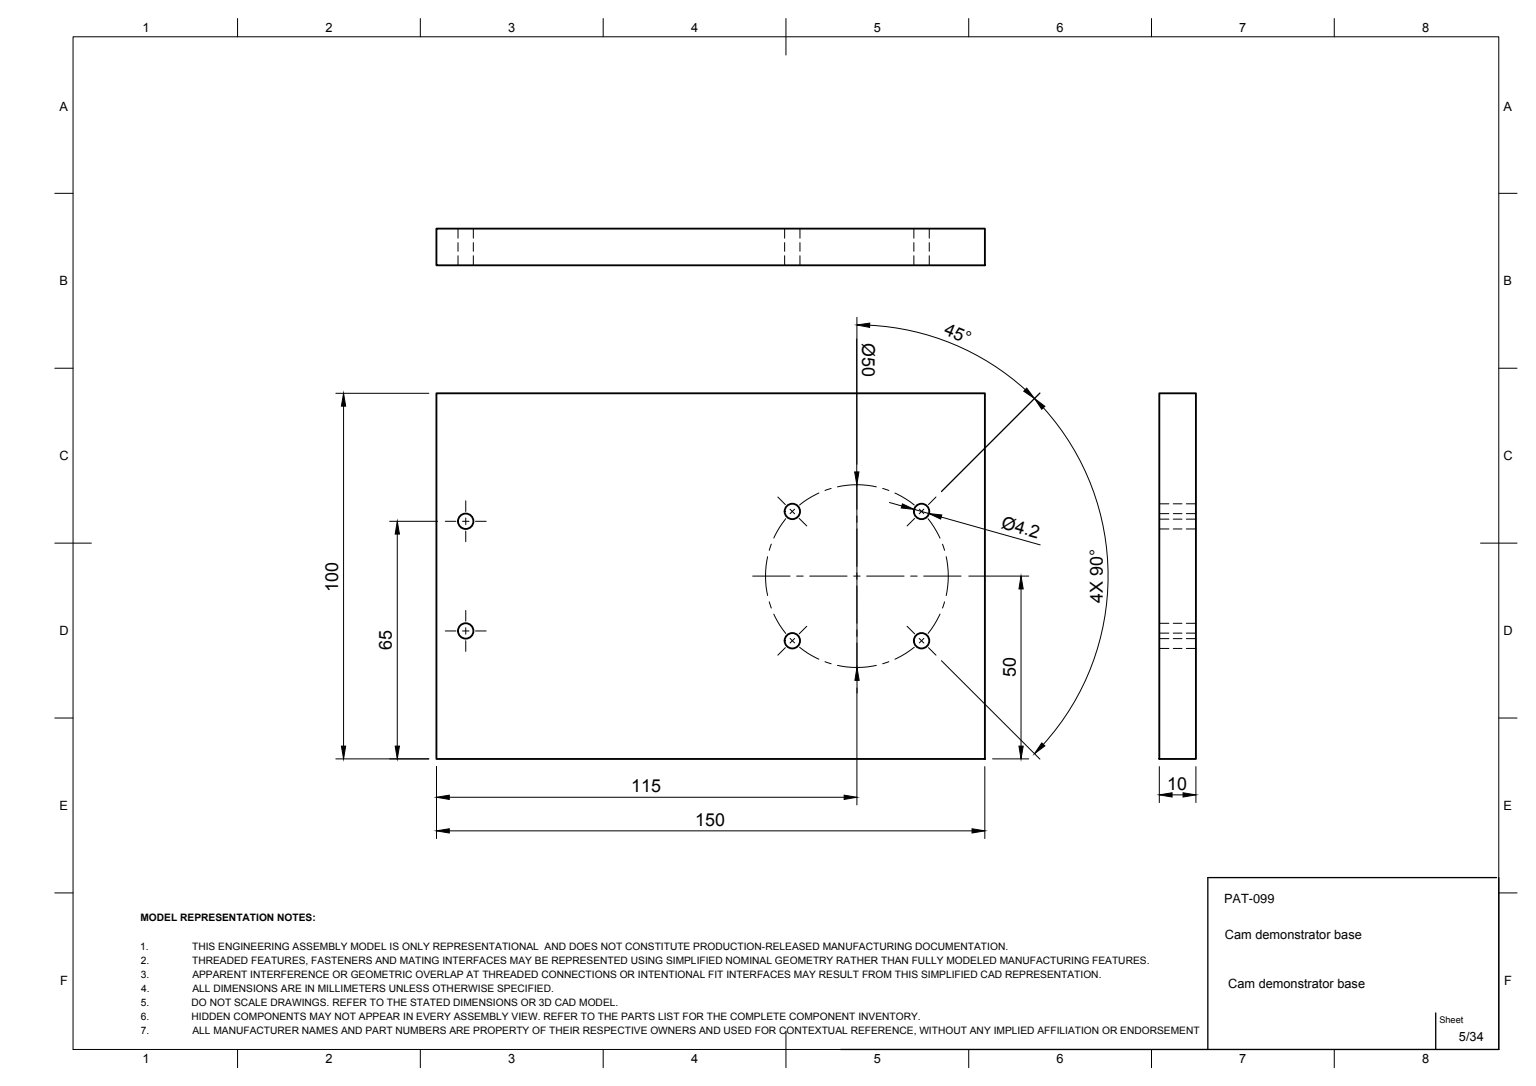
ISO-10303-21;
HEADER;
/* Generated by software containing ST-Developer
 * from STEP Tools, Inc. (www.steptools.com) 
 */

FILE_DESCRIPTION(
/* description */ ('PAT-099'),
/* implementation_level */ '2;1');

FILE_NAME(
/* name */ 'Cam demonstrator base.step',
/* time_stamp */ '2026-10-29T17:25:42-07:00',
/* author */ (''),
/* organization */ (''),
/* preprocessor_version */ 'ST-DEVELOPER v20.2',
/* originating_system */ 'Autodesk Translation Framework v15.17.0.0',
/* authorisation */ '');

FILE_SCHEMA (('AUTOMOTIVE_DESIGN { 1 0 10303 214 3 1 1 }'));
ENDSEC;

DATA;
#10=MECHANICAL_DESIGN_GEOMETRIC_PRESENTATION_REPRESENTATION('',(#337),#11035);
#287=SHAPE_REPRESENTATION_RELATIONSHIP('SRR','None',#11155,#312);
#312=ADVANCED_BREP_SHAPE_REPRESENTATION('',(#370),#11005);
#337=STYLED_ITEM('',(#11365),#370);
#370=MANIFOLD_SOLID_BREP('Body1',#4705);
#401=FACE_BOUND('',#951,.T.);
#402=FACE_BOUND('',#952,.T.);
#403=FACE_BOUND('',#953,.T.);
#404=FACE_BOUND('',#954,.T.);
#405=FACE_BOUND('',#955,.T.);
#406=FACE_BOUND('',#956,.T.);
#407=FACE_BOUND('',#958,.T.);
#408=FACE_BOUND('',#959,.T.);
#409=FACE_BOUND('',#960,.T.);
#410=FACE_BOUND('',#961,.T.);
#411=FACE_BOUND('',#962,.T.);
#412=FACE_BOUND('',#963,.T.);
#523=PLANE('',#5037);
#524=PLANE('',#5038);
#525=PLANE('',#5039);
#526=PLANE('',#5040);
#527=PLANE('',#5041);
#528=PLANE('',#5042);
#659=FACE_OUTER_BOUND('',#940,.T.);
#660=FACE_OUTER_BOUND('',#941,.T.);
#661=FACE_OUTER_BOUND('',#942,.T.);
#662=FACE_OUTER_BOUND('',#943,.T.);
#663=FACE_OUTER_BOUND('',#944,.T.);
#664=FACE_OUTER_BOUND('',#945,.T.);
#665=FACE_OUTER_BOUND('',#946,.T.);
#666=FACE_OUTER_BOUND('',#947,.T.);
#667=FACE_OUTER_BOUND('',#948,.T.);
#668=FACE_OUTER_BOUND('',#949,.T.);
#669=FACE_OUTER_BOUND('',#950,.T.);
#670=FACE_OUTER_BOUND('',#957,.T.);
#940=EDGE_LOOP('',(#3131,#3132,#3133,#3134));
#941=EDGE_LOOP('',(#3135,#3136,#3137,#3138));
#942=EDGE_LOOP('',(#3139,#3140,#3141,#3142));
#943=EDGE_LOOP('',(#3143,#3144,#3145,#3146));
#944=EDGE_LOOP('',(#3147,#3148,#3149,#3150));
#945=EDGE_LOOP('',(#3151,#3152,#3153,#3154));
#946=EDGE_LOOP('',(#3155,#3156,#3157,#3158));
#947=EDGE_LOOP('',(#3159,#3160,#3161,#3162));
#948=EDGE_LOOP('',(#3163,#3164,#3165,#3166));
#949=EDGE_LOOP('',(#3167,#3168,#3169,#3170));
#950=EDGE_LOOP('',(#3171,#3172,#3173,#3174));
#951=EDGE_LOOP('',(#3175));
#952=EDGE_LOOP('',(#3176));
#953=EDGE_LOOP('',(#3177));
#954=EDGE_LOOP('',(#3178));
#955=EDGE_LOOP('',(#3179));
#956=EDGE_LOOP('',(#3180));
#957=EDGE_LOOP('',(#3181,#3182,#3183,#3184));
#958=EDGE_LOOP('',(#3185));
#959=EDGE_LOOP('',(#3186));
#960=EDGE_LOOP('',(#3187));
#961=EDGE_LOOP('',(#3188));
#962=EDGE_LOOP('',(#3189));
#963=EDGE_LOOP('',(#3190));
#1343=LINE('',#7231,#1595);
#1344=LINE('',#7237,#1596);
#1345=LINE('',#7243,#1597);
#1346=LINE('',#7249,#1598);
#1347=LINE('',#7255,#1599);
#1348=LINE('',#7261,#1600);
#1349=LINE('',#7266,#1601);
#1350=LINE('',#7268,#1602);
#1351=LINE('',#7270,#1603);
#1352=LINE('',#7271,#1604);
#1353=LINE('',#7274,#1605);
#1354=LINE('',#7276,#1606);
#1355=LINE('',#7277,#1607);
#1356=LINE('',#7280,#1608);
#1357=LINE('',#7282,#1609);
#1358=LINE('',#7283,#1610);
#1359=LINE('',#7285,#1611);
#1360=LINE('',#7286,#1612);
#1595=VECTOR('',#5678,0.210000000000001);
#1596=VECTOR('',#5685,0.210000000000001);
#1597=VECTOR('',#5692,0.21);
#1598=VECTOR('',#5699,0.21);
#1599=VECTOR('',#5706,0.21);
#1600=VECTOR('',#5713,0.21);
#1601=VECTOR('',#5718,1.);
#1602=VECTOR('',#5719,1.);
#1603=VECTOR('',#5720,1.);
#1604=VECTOR('',#5721,1.);
#1605=VECTOR('',#5724,1.);
#1606=VECTOR('',#5725,1.);
#1607=VECTOR('',#5726,1.);
#1608=VECTOR('',#5729,1.);
#1609=VECTOR('',#5730,1.);
#1610=VECTOR('',#5731,1.);
#1611=VECTOR('',#5734,1.);
#1612=VECTOR('',#5735,1.);
#1847=CIRCLE('',#5020,0.210000000000001);
#1848=CIRCLE('',#5021,0.210000000000001);
#1849=CIRCLE('',#5023,0.210000000000001);
#1850=CIRCLE('',#5024,0.210000000000001);
#1851=CIRCLE('',#5026,0.21);
#1852=CIRCLE('',#5027,0.21);
#1853=CIRCLE('',#5029,0.21);
#1854=CIRCLE('',#5030,0.21);
#1855=CIRCLE('',#5032,0.21);
#1856=CIRCLE('',#5033,0.21);
#1857=CIRCLE('',#5035,0.21);
#1858=CIRCLE('',#5036,0.21);
#2138=VERTEX_POINT('',#7228);
#2139=VERTEX_POINT('',#7230);
#2140=VERTEX_POINT('',#7234);
#2141=VERTEX_POINT('',#7236);
#2142=VERTEX_POINT('',#7240);
#2143=VERTEX_POINT('',#7242);
#2144=VERTEX_POINT('',#7246);
#2145=VERTEX_POINT('',#7248);
#2146=VERTEX_POINT('',#7252);
#2147=VERTEX_POINT('',#7254);
#2148=VERTEX_POINT('',#7258);
#2149=VERTEX_POINT('',#7260);
#2150=VERTEX_POINT('',#7264);
#2151=VERTEX_POINT('',#7265);
#2152=VERTEX_POINT('',#7267);
#2153=VERTEX_POINT('',#7269);
#2154=VERTEX_POINT('',#7273);
#2155=VERTEX_POINT('',#7275);
#2156=VERTEX_POINT('',#7279);
#2157=VERTEX_POINT('',#7281);
#2542=EDGE_CURVE('',#2138,#2138,#1847,.T.);
#2543=EDGE_CURVE('',#2138,#2139,#1343,.T.);
#2544=EDGE_CURVE('',#2139,#2139,#1848,.T.);
#2545=EDGE_CURVE('',#2140,#2140,#1849,.T.);
#2546=EDGE_CURVE('',#2140,#2141,#1344,.T.);
#2547=EDGE_CURVE('',#2141,#2141,#1850,.T.);
#2548=EDGE_CURVE('',#2142,#2142,#1851,.T.);
#2549=EDGE_CURVE('',#2142,#2143,#1345,.T.);
#2550=EDGE_CURVE('',#2143,#2143,#1852,.T.);
#2551=EDGE_CURVE('',#2144,#2144,#1853,.T.);
#2552=EDGE_CURVE('',#2144,#2145,#1346,.T.);
#2553=EDGE_CURVE('',#2145,#2145,#1854,.T.);
#2554=EDGE_CURVE('',#2146,#2146,#1855,.T.);
#2555=EDGE_CURVE('',#2146,#2147,#1347,.T.);
#2556=EDGE_CURVE('',#2147,#2147,#1856,.T.);
#2557=EDGE_CURVE('',#2148,#2148,#1857,.T.);
#2558=EDGE_CURVE('',#2148,#2149,#1348,.T.);
#2559=EDGE_CURVE('',#2149,#2149,#1858,.T.);
#2560=EDGE_CURVE('',#2150,#2151,#1349,.T.);
#2561=EDGE_CURVE('',#2151,#2152,#1350,.T.);
#2562=EDGE_CURVE('',#2153,#2152,#1351,.T.);
#2563=EDGE_CURVE('',#2150,#2153,#1352,.T.);
#2564=EDGE_CURVE('',#2154,#2150,#1353,.T.);
#2565=EDGE_CURVE('',#2155,#2153,#1354,.T.);
#2566=EDGE_CURVE('',#2154,#2155,#1355,.T.);
#2567=EDGE_CURVE('',#2156,#2154,#1356,.T.);
#2568=EDGE_CURVE('',#2157,#2155,#1357,.T.);
#2569=EDGE_CURVE('',#2156,#2157,#1358,.T.);
#2570=EDGE_CURVE('',#2151,#2156,#1359,.T.);
#2571=EDGE_CURVE('',#2152,#2157,#1360,.T.);
#3131=ORIENTED_EDGE('',*,*,#2542,.F.);
#3132=ORIENTED_EDGE('',*,*,#2543,.T.);
#3133=ORIENTED_EDGE('',*,*,#2544,.F.);
#3134=ORIENTED_EDGE('',*,*,#2543,.F.);
#3135=ORIENTED_EDGE('',*,*,#2545,.F.);
#3136=ORIENTED_EDGE('',*,*,#2546,.T.);
#3137=ORIENTED_EDGE('',*,*,#2547,.F.);
#3138=ORIENTED_EDGE('',*,*,#2546,.F.);
#3139=ORIENTED_EDGE('',*,*,#2548,.F.);
#3140=ORIENTED_EDGE('',*,*,#2549,.T.);
#3141=ORIENTED_EDGE('',*,*,#2550,.F.);
#3142=ORIENTED_EDGE('',*,*,#2549,.F.);
#3143=ORIENTED_EDGE('',*,*,#2551,.F.);
#3144=ORIENTED_EDGE('',*,*,#2552,.T.);
#3145=ORIENTED_EDGE('',*,*,#2553,.F.);
#3146=ORIENTED_EDGE('',*,*,#2552,.F.);
#3147=ORIENTED_EDGE('',*,*,#2554,.F.);
#3148=ORIENTED_EDGE('',*,*,#2555,.T.);
#3149=ORIENTED_EDGE('',*,*,#2556,.F.);
#3150=ORIENTED_EDGE('',*,*,#2555,.F.);
#3151=ORIENTED_EDGE('',*,*,#2557,.F.);
#3152=ORIENTED_EDGE('',*,*,#2558,.T.);
#3153=ORIENTED_EDGE('',*,*,#2559,.F.);
#3154=ORIENTED_EDGE('',*,*,#2558,.F.);
#3155=ORIENTED_EDGE('',*,*,#2560,.T.);
#3156=ORIENTED_EDGE('',*,*,#2561,.T.);
#3157=ORIENTED_EDGE('',*,*,#2562,.F.);
#3158=ORIENTED_EDGE('',*,*,#2563,.F.);
#3159=ORIENTED_EDGE('',*,*,#2564,.T.);
#3160=ORIENTED_EDGE('',*,*,#2563,.T.);
#3161=ORIENTED_EDGE('',*,*,#2565,.F.);
#3162=ORIENTED_EDGE('',*,*,#2566,.F.);
#3163=ORIENTED_EDGE('',*,*,#2567,.T.);
#3164=ORIENTED_EDGE('',*,*,#2566,.T.);
#3165=ORIENTED_EDGE('',*,*,#2568,.F.);
#3166=ORIENTED_EDGE('',*,*,#2569,.F.);
#3167=ORIENTED_EDGE('',*,*,#2570,.T.);
#3168=ORIENTED_EDGE('',*,*,#2569,.T.);
#3169=ORIENTED_EDGE('',*,*,#2571,.F.);
#3170=ORIENTED_EDGE('',*,*,#2561,.F.);
#3171=ORIENTED_EDGE('',*,*,#2571,.T.);
#3172=ORIENTED_EDGE('',*,*,#2568,.T.);
#3173=ORIENTED_EDGE('',*,*,#2565,.T.);
#3174=ORIENTED_EDGE('',*,*,#2562,.T.);
#3175=ORIENTED_EDGE('',*,*,#2544,.T.);
#3176=ORIENTED_EDGE('',*,*,#2547,.T.);
#3177=ORIENTED_EDGE('',*,*,#2550,.T.);
#3178=ORIENTED_EDGE('',*,*,#2553,.T.);
#3179=ORIENTED_EDGE('',*,*,#2556,.T.);
#3180=ORIENTED_EDGE('',*,*,#2559,.T.);
#3181=ORIENTED_EDGE('',*,*,#2570,.F.);
#3182=ORIENTED_EDGE('',*,*,#2560,.F.);
#3183=ORIENTED_EDGE('',*,*,#2564,.F.);
#3184=ORIENTED_EDGE('',*,*,#2567,.F.);
#3185=ORIENTED_EDGE('',*,*,#2542,.T.);
#3186=ORIENTED_EDGE('',*,*,#2545,.T.);
#3187=ORIENTED_EDGE('',*,*,#2548,.T.);
#3188=ORIENTED_EDGE('',*,*,#2551,.T.);
#3189=ORIENTED_EDGE('',*,*,#2554,.T.);
#3190=ORIENTED_EDGE('',*,*,#2557,.T.);
#4309=CYLINDRICAL_SURFACE('',#5019,0.210000000000001);
#4310=CYLINDRICAL_SURFACE('',#5022,0.210000000000001);
#4311=CYLINDRICAL_SURFACE('',#5025,0.21);
#4312=CYLINDRICAL_SURFACE('',#5028,0.21);
#4313=CYLINDRICAL_SURFACE('',#5031,0.21);
#4314=CYLINDRICAL_SURFACE('',#5034,0.21);
#4424=ADVANCED_FACE('',(#659),#4309,.F.);
#4425=ADVANCED_FACE('',(#660),#4310,.F.);
#4426=ADVANCED_FACE('',(#661),#4311,.F.);
#4427=ADVANCED_FACE('',(#662),#4312,.F.);
#4428=ADVANCED_FACE('',(#663),#4313,.F.);
#4429=ADVANCED_FACE('',(#664),#4314,.F.);
#4430=ADVANCED_FACE('',(#665),#523,.T.);
#4431=ADVANCED_FACE('',(#666),#524,.T.);
#4432=ADVANCED_FACE('',(#667),#525,.T.);
#4433=ADVANCED_FACE('',(#668),#526,.T.);
#4434=ADVANCED_FACE('',(#669,#401,#402,#403,#404,#405,#406),#527,.T.);
#4435=ADVANCED_FACE('',(#670,#407,#408,#409,#410,#411,#412),#528,.F.);
#4705=CLOSED_SHELL('',(#4424,#4425,#4426,#4427,#4428,#4429,#4430,#4431,
#4432,#4433,#4434,#4435));
#5018=AXIS2_PLACEMENT_3D('',#7226,#5672,#5673);
#5019=AXIS2_PLACEMENT_3D('',#7227,#5674,#5675);
#5020=AXIS2_PLACEMENT_3D('',#7229,#5676,#5677);
#5021=AXIS2_PLACEMENT_3D('',#7232,#5679,#5680);
#5022=AXIS2_PLACEMENT_3D('',#7233,#5681,#5682);
#5023=AXIS2_PLACEMENT_3D('',#7235,#5683,#5684);
#5024=AXIS2_PLACEMENT_3D('',#7238,#5686,#5687);
#5025=AXIS2_PLACEMENT_3D('',#7239,#5688,#5689);
#5026=AXIS2_PLACEMENT_3D('',#7241,#5690,#5691);
#5027=AXIS2_PLACEMENT_3D('',#7244,#5693,#5694);
#5028=AXIS2_PLACEMENT_3D('',#7245,#5695,#5696);
#5029=AXIS2_PLACEMENT_3D('',#7247,#5697,#5698);
#5030=AXIS2_PLACEMENT_3D('',#7250,#5700,#5701);
#5031=AXIS2_PLACEMENT_3D('',#7251,#5702,#5703);
#5032=AXIS2_PLACEMENT_3D('',#7253,#5704,#5705);
#5033=AXIS2_PLACEMENT_3D('',#7256,#5707,#5708);
#5034=AXIS2_PLACEMENT_3D('',#7257,#5709,#5710);
#5035=AXIS2_PLACEMENT_3D('',#7259,#5711,#5712);
#5036=AXIS2_PLACEMENT_3D('',#7262,#5714,#5715);
#5037=AXIS2_PLACEMENT_3D('',#7263,#5716,#5717);
#5038=AXIS2_PLACEMENT_3D('',#7272,#5722,#5723);
#5039=AXIS2_PLACEMENT_3D('',#7278,#5727,#5728);
#5040=AXIS2_PLACEMENT_3D('',#7284,#5732,#5733);
#5041=AXIS2_PLACEMENT_3D('',#7287,#5736,#5737);
#5042=AXIS2_PLACEMENT_3D('',#7288,#5738,#5739);
#5672=DIRECTION('axis',(0.,0.,1.));
#5673=DIRECTION('refdir',(1.,0.,0.));
#5674=DIRECTION('center_axis',(0.,0.,1.));
#5675=DIRECTION('ref_axis',(1.,0.,0.));
#5676=DIRECTION('center_axis',(0.,0.,1.));
#5677=DIRECTION('ref_axis',(1.,0.,0.));
#5678=DIRECTION('',(0.,0.,1.));
#5679=DIRECTION('center_axis',(0.,0.,-1.));
#5680=DIRECTION('ref_axis',(1.,0.,0.));
#5681=DIRECTION('center_axis',(0.,0.,1.));
#5682=DIRECTION('ref_axis',(1.,0.,0.));
#5683=DIRECTION('center_axis',(0.,0.,1.));
#5684=DIRECTION('ref_axis',(1.,0.,0.));
#5685=DIRECTION('',(0.,0.,1.));
#5686=DIRECTION('center_axis',(0.,0.,-1.));
#5687=DIRECTION('ref_axis',(1.,0.,0.));
#5688=DIRECTION('center_axis',(0.,0.,1.));
#5689=DIRECTION('ref_axis',(1.,0.,0.));
#5690=DIRECTION('center_axis',(0.,0.,1.));
#5691=DIRECTION('ref_axis',(1.,0.,0.));
#5692=DIRECTION('',(0.,0.,1.));
#5693=DIRECTION('center_axis',(0.,0.,-1.));
#5694=DIRECTION('ref_axis',(1.,0.,0.));
#5695=DIRECTION('center_axis',(0.,0.,1.));
#5696=DIRECTION('ref_axis',(1.,0.,0.));
#5697=DIRECTION('center_axis',(0.,0.,1.));
#5698=DIRECTION('ref_axis',(1.,0.,0.));
#5699=DIRECTION('',(0.,0.,1.));
#5700=DIRECTION('center_axis',(0.,0.,-1.));
#5701=DIRECTION('ref_axis',(1.,0.,0.));
#5702=DIRECTION('center_axis',(0.,0.,1.));
#5703=DIRECTION('ref_axis',(1.,0.,0.));
#5704=DIRECTION('center_axis',(0.,0.,1.));
#5705=DIRECTION('ref_axis',(1.,0.,0.));
#5706=DIRECTION('',(0.,0.,1.));
#5707=DIRECTION('center_axis',(0.,0.,-1.));
#5708=DIRECTION('ref_axis',(1.,0.,0.));
#5709=DIRECTION('center_axis',(0.,0.,1.));
#5710=DIRECTION('ref_axis',(1.,0.,0.));
#5711=DIRECTION('center_axis',(0.,0.,1.));
#5712=DIRECTION('ref_axis',(1.,0.,0.));
#5713=DIRECTION('',(0.,0.,1.));
#5714=DIRECTION('center_axis',(0.,0.,-1.));
#5715=DIRECTION('ref_axis',(1.,0.,0.));
#5716=DIRECTION('center_axis',(0.,1.,0.));
#5717=DIRECTION('ref_axis',(-1.,0.,0.));
#5718=DIRECTION('',(-1.,0.,0.));
#5719=DIRECTION('',(0.,0.,1.));
#5720=DIRECTION('',(-1.,0.,0.));
#5721=DIRECTION('',(0.,0.,1.));
#5722=DIRECTION('center_axis',(1.,0.,0.));
#5723=DIRECTION('ref_axis',(0.,1.,0.));
#5724=DIRECTION('',(0.,1.,0.));
#5725=DIRECTION('',(0.,1.,0.));
#5726=DIRECTION('',(0.,0.,1.));
#5727=DIRECTION('center_axis',(0.,-1.,0.));
#5728=DIRECTION('ref_axis',(1.,0.,0.));
#5729=DIRECTION('',(1.,0.,0.));
#5730=DIRECTION('',(1.,0.,0.));
#5731=DIRECTION('',(0.,0.,1.));
#5732=DIRECTION('center_axis',(-1.,0.,0.));
#5733=DIRECTION('ref_axis',(0.,-1.,0.));
#5734=DIRECTION('',(0.,-1.,0.));
#5735=DIRECTION('',(0.,-1.,0.));
#5736=DIRECTION('center_axis',(0.,0.,1.));
#5737=DIRECTION('ref_axis',(1.,0.,0.));
#5738=DIRECTION('center_axis',(0.,0.,1.));
#5739=DIRECTION('ref_axis',(1.,0.,0.));
#7226=CARTESIAN_POINT('',(0.,0.,0.));
#7227=CARTESIAN_POINT('Origin',(10.7,1.5,-0.1));
#7228=CARTESIAN_POINT('',(10.49,1.5,0.));
#7229=CARTESIAN_POINT('Origin',(10.7,1.5,0.));
#7230=CARTESIAN_POINT('',(10.49,1.5,1.));
#7231=CARTESIAN_POINT('',(10.49,1.5,-0.1));
#7232=CARTESIAN_POINT('Origin',(10.7,1.5,1.));
#7233=CARTESIAN_POINT('Origin',(10.7,-1.5,-0.1));
#7234=CARTESIAN_POINT('',(10.49,-1.5,0.));
#7235=CARTESIAN_POINT('Origin',(10.7,-1.5,0.));
#7236=CARTESIAN_POINT('',(10.49,-1.5,1.));
#7237=CARTESIAN_POINT('',(10.49,-1.5,-0.1));
#7238=CARTESIAN_POINT('Origin',(10.7,-1.5,1.));
#7239=CARTESIAN_POINT('Origin',(1.76776695296637,-1.76776695296637,-0.1));
#7240=CARTESIAN_POINT('',(1.55776695296637,-1.76776695296637,0.));
#7241=CARTESIAN_POINT('Origin',(1.76776695296637,-1.76776695296637,0.));
#7242=CARTESIAN_POINT('',(1.55776695296637,-1.76776695296637,1.));
#7243=CARTESIAN_POINT('',(1.55776695296637,-1.76776695296637,-0.1));
#7244=CARTESIAN_POINT('Origin',(1.76776695296637,-1.76776695296637,1.));
#7245=CARTESIAN_POINT('Origin',(-1.76776695296637,-1.76776695296637,-0.1));
#7246=CARTESIAN_POINT('',(-1.97776695296637,-1.76776695296637,0.));
#7247=CARTESIAN_POINT('Origin',(-1.76776695296637,-1.76776695296637,0.));
#7248=CARTESIAN_POINT('',(-1.97776695296637,-1.76776695296637,1.));
#7249=CARTESIAN_POINT('',(-1.97776695296637,-1.76776695296637,-0.1));
#7250=CARTESIAN_POINT('Origin',(-1.76776695296637,-1.76776695296637,1.));
#7251=CARTESIAN_POINT('Origin',(-1.76776695296637,1.76776695296637,-0.1));
#7252=CARTESIAN_POINT('',(-1.97776695296637,1.76776695296637,0.));
#7253=CARTESIAN_POINT('Origin',(-1.76776695296637,1.76776695296637,0.));
#7254=CARTESIAN_POINT('',(-1.97776695296637,1.76776695296637,1.));
#7255=CARTESIAN_POINT('',(-1.97776695296637,1.76776695296637,-0.1));
#7256=CARTESIAN_POINT('Origin',(-1.76776695296637,1.76776695296637,1.));
#7257=CARTESIAN_POINT('Origin',(1.76776695296637,1.76776695296637,-0.1));
#7258=CARTESIAN_POINT('',(1.55776695296637,1.76776695296637,0.));
#7259=CARTESIAN_POINT('Origin',(1.76776695296637,1.76776695296637,0.));
#7260=CARTESIAN_POINT('',(1.55776695296637,1.76776695296637,1.));
#7261=CARTESIAN_POINT('',(1.55776695296637,1.76776695296637,-0.1));
#7262=CARTESIAN_POINT('Origin',(1.76776695296637,1.76776695296637,1.));
#7263=CARTESIAN_POINT('Origin',(11.5,5.,0.));
#7264=CARTESIAN_POINT('',(11.5,5.,0.));
#7265=CARTESIAN_POINT('',(-3.5,5.,0.));
#7266=CARTESIAN_POINT('',(11.5,5.,0.));
#7267=CARTESIAN_POINT('',(-3.5,5.,1.));
#7268=CARTESIAN_POINT('',(-3.5,5.,0.));
#7269=CARTESIAN_POINT('',(11.5,5.,1.));
#7270=CARTESIAN_POINT('',(11.5,5.,1.));
#7271=CARTESIAN_POINT('',(11.5,5.,0.));
#7272=CARTESIAN_POINT('Origin',(11.5,-5.,0.));
#7273=CARTESIAN_POINT('',(11.5,-5.,0.));
#7274=CARTESIAN_POINT('',(11.5,-5.,0.));
#7275=CARTESIAN_POINT('',(11.5,-5.,1.));
#7276=CARTESIAN_POINT('',(11.5,-5.,1.));
#7277=CARTESIAN_POINT('',(11.5,-5.,0.));
#7278=CARTESIAN_POINT('Origin',(-3.5,-5.,0.));
#7279=CARTESIAN_POINT('',(-3.5,-5.,0.));
#7280=CARTESIAN_POINT('',(-3.5,-5.,0.));
#7281=CARTESIAN_POINT('',(-3.5,-5.,1.));
#7282=CARTESIAN_POINT('',(-3.5,-5.,1.));
#7283=CARTESIAN_POINT('',(-3.5,-5.,0.));
#7284=CARTESIAN_POINT('Origin',(-3.5,5.,0.));
#7285=CARTESIAN_POINT('',(-3.5,5.,0.));
#7286=CARTESIAN_POINT('',(-3.5,5.,1.));
#7287=CARTESIAN_POINT('Origin',(4.,0.,1.));
#7288=CARTESIAN_POINT('Origin',(4.,0.,0.));
#10972=UNCERTAINTY_MEASURE_WITH_UNIT(LENGTH_MEASURE(0.001),#11036,
'DISTANCE_ACCURACY_VALUE',
'Maximum model space distance between geometric entities at asserted c
onnectivities');
#11002=UNCERTAINTY_MEASURE_WITH_UNIT(LENGTH_MEASURE(0.001),#11036,
'DISTANCE_ACCURACY_VALUE',
'Maximum model space distance between geometric entities at asserted c
onnectivities');
#11005=(
GEOMETRIC_REPRESENTATION_CONTEXT(3)
GLOBAL_UNCERTAINTY_ASSIGNED_CONTEXT((#10972))
GLOBAL_UNIT_ASSIGNED_CONTEXT((#11036,#11038,#11039))
REPRESENTATION_CONTEXT('','3D')
);
#11035=(
GEOMETRIC_REPRESENTATION_CONTEXT(3)
GLOBAL_UNCERTAINTY_ASSIGNED_CONTEXT((#11002))
GLOBAL_UNIT_ASSIGNED_CONTEXT((#11036,#11038,#11039))
REPRESENTATION_CONTEXT('','3D')
);
#11036=(
LENGTH_UNIT()
NAMED_UNIT(*)
SI_UNIT(.CENTI.,.METRE.)
);
#11038=(
NAMED_UNIT(*)
PLANE_ANGLE_UNIT()
SI_UNIT($,.RADIAN.)
);
#11039=(
NAMED_UNIT(*)
SI_UNIT($,.STERADIAN.)
SOLID_ANGLE_UNIT()
);
#11042=SHAPE_DEFINITION_REPRESENTATION(#11074,#11155);
#11074=PRODUCT_DEFINITION_SHAPE('',$,#11188);
#11155=SHAPE_REPRESENTATION('',(#5018),#11005);
#11185=PRODUCT_DEFINITION_CONTEXT('part definition',#11283,'design');
#11188=PRODUCT_DEFINITION('Cam demonstrator base',
'Cam demonstrator base',#11220,#11185);
#11220=PRODUCT_DEFINITION_FORMATION('',$,#11287);
#11283=APPLICATION_CONTEXT(
'Core Data for Automotive Mechanical Design Process');
#11284=PRODUCT_CONTEXT('part definition',#11283,'mechanical');
#11287=PRODUCT('Cam demonstrator base','Cam demonstrator base',
'Cam demonstrator base',(#11284));
#11359=COLOUR_RGB('Dark Blue',0.08,0.2,0.34);
#11360=FILL_AREA_STYLE_COLOUR('',#11359);
#11361=FILL_AREA_STYLE('',(#11360));
#11362=SURFACE_STYLE_FILL_AREA(#11361);
#11363=SURFACE_SIDE_STYLE('',(#11362));
#11364=SURFACE_STYLE_USAGE(.BOTH.,#11363);
#11365=PRESENTATION_STYLE_ASSIGNMENT((#11364));
ENDSEC;
END-ISO-10303-21;
